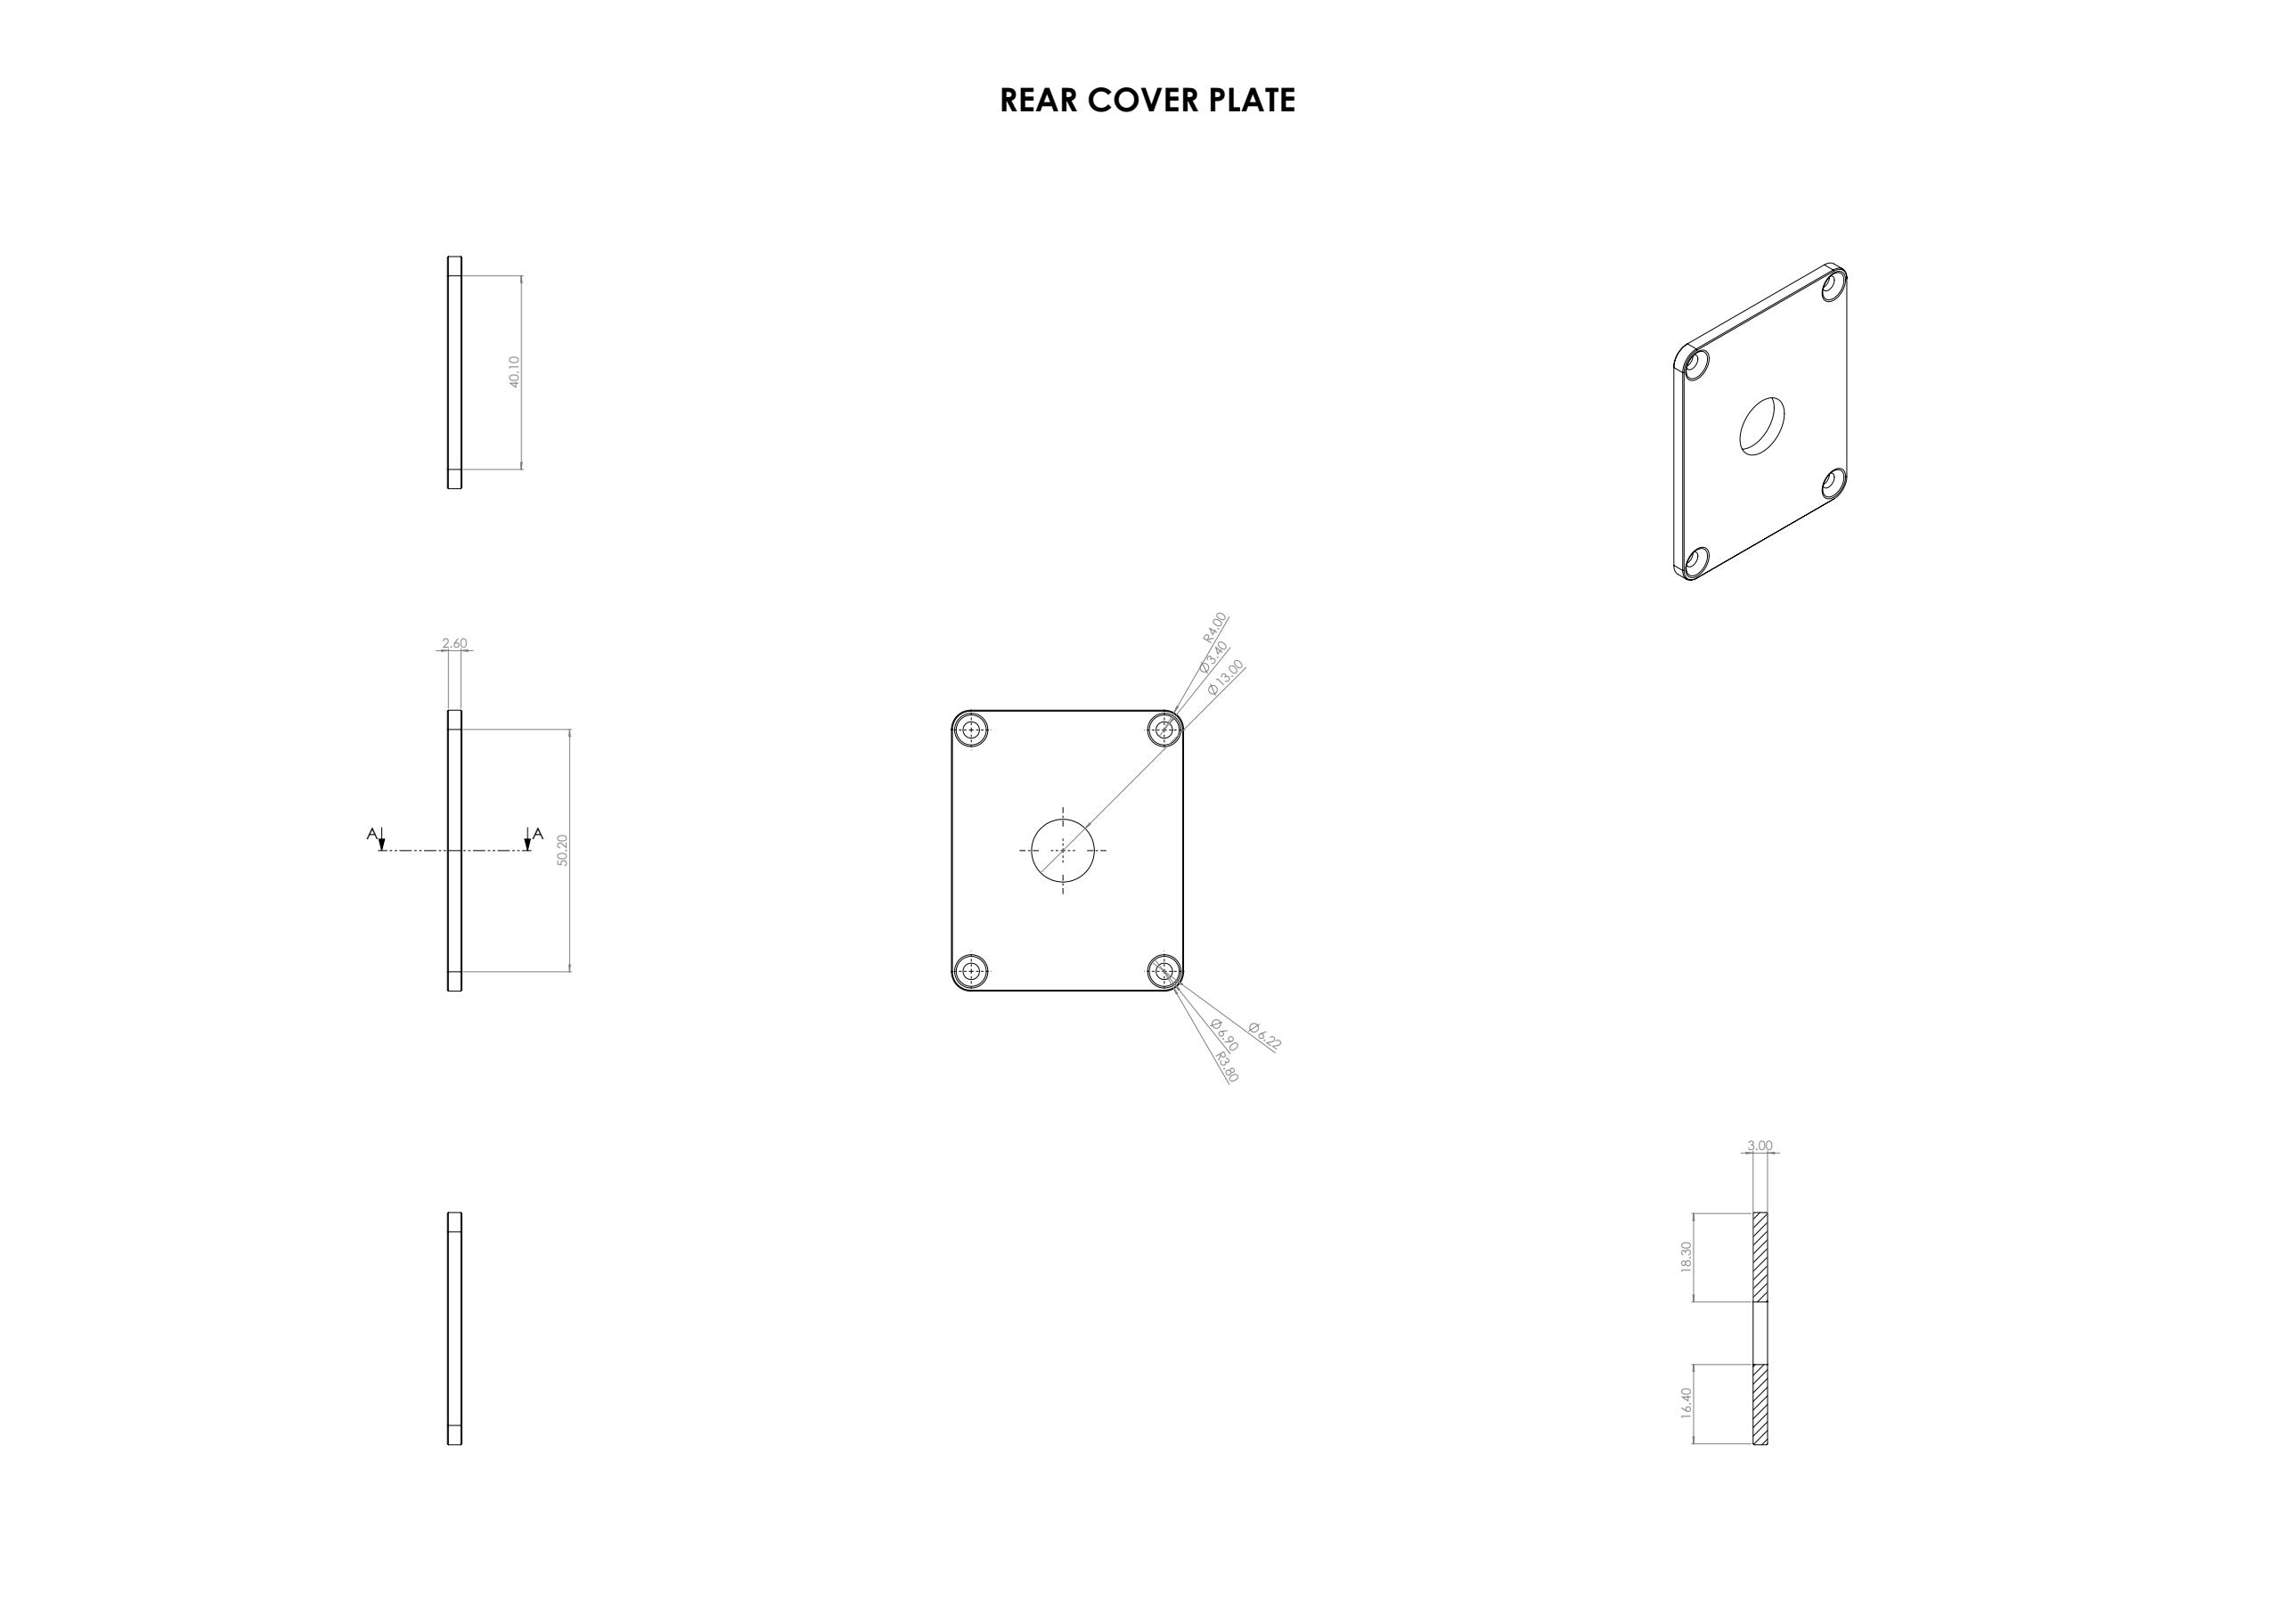
ISO-10303-21;
HEADER;
/* Generated by software containing ST-Developer
 * from STEP Tools, Inc. (www.steptools.com) 
 */

FILE_DESCRIPTION(
/* description */ (''),
/* implementation_level */ '2;1');

FILE_NAME(
/* name */ '07_Rear_Cover_Plate.step',
/* time_stamp */ '2026-10-21T01:59:45-07:00',
/* author */ (''),
/* organization */ (''),
/* preprocessor_version */ 'ST-DEVELOPER v20.2',
/* originating_system */ 'Autodesk Translation Framework v15.15.0.0',
/* authorisation */ '');

FILE_SCHEMA (('AUTOMOTIVE_DESIGN { 1 0 10303 214 3 1 1 }'));
ENDSEC;

DATA;
#10=MECHANICAL_DESIGN_GEOMETRIC_PRESENTATION_REPRESENTATION('',(#466),#18281);
#392=CONICAL_SURFACE('',#9472,3.9,0.78539816339746);
#393=CONICAL_SURFACE('',#9476,3.9,0.785398163397461);
#394=CONICAL_SURFACE('',#9480,3.9,0.785398163397455);
#395=CONICAL_SURFACE('',#9484,3.9,0.785398163397455);
#396=CONICAL_SURFACE('',#9499,3.27928932188134,1.17809724509612);
#397=CONICAL_SURFACE('',#9511,2.475,0.785398163397451);
#398=CONICAL_SURFACE('',#9514,3.9,0.785398163397461);
#399=CONICAL_SURFACE('',#9517,3.9,0.785398163397455);
#400=CONICAL_SURFACE('',#9519,3.9,0.785398163397455);
#401=CONICAL_SURFACE('',#9521,3.9,0.78539816339746);
#402=CONICAL_SURFACE('',#9526,3.27928932188135,1.17809724509617);
#403=CONICAL_SURFACE('',#9528,2.475,0.78539816339745);
#404=CONICAL_SURFACE('',#9530,3.27928932188135,1.17809724509617);
#405=CONICAL_SURFACE('',#9532,2.475,0.78539816339745);
#406=CONICAL_SURFACE('',#9534,3.27928932188134,1.17809724509612);
#407=CONICAL_SURFACE('',#9536,2.475,0.785398163397451);
#440=SHAPE_REPRESENTATION_RELATIONSHIP('SRR','None',#18342,#453);
#453=ADVANCED_BREP_SHAPE_REPRESENTATION('',(#484),#18271);
#466=STYLED_ITEM('',(#18467),#484);
#484=MANIFOLD_SOLID_BREP('Body1',#9088);
#508=CYLINDRICAL_SURFACE('',#9487,4.);
#509=CYLINDRICAL_SURFACE('',#9490,4.);
#510=CYLINDRICAL_SURFACE('',#9524,4.);
#511=CYLINDRICAL_SURFACE('',#9538,1.7);
#512=CYLINDRICAL_SURFACE('',#9539,1.7);
#513=CYLINDRICAL_SURFACE('',#9540,1.7);
#514=CYLINDRICAL_SURFACE('',#9541,1.7);
#515=CYLINDRICAL_SURFACE('',#9542,6.5);
#516=CYLINDRICAL_SURFACE('',#9543,4.);
#598=FACE_BOUND('',#1602,.T.);
#599=FACE_BOUND('',#1603,.T.);
#600=FACE_BOUND('',#1604,.T.);
#601=FACE_BOUND('',#1605,.T.);
#602=FACE_BOUND('',#1606,.T.);
#603=FACE_BOUND('',#1609,.T.);
#604=FACE_BOUND('',#1610,.T.);
#605=FACE_BOUND('',#1611,.T.);
#606=FACE_BOUND('',#1612,.T.);
#607=FACE_BOUND('',#1613,.T.);
#679=CIRCLE('',#9473,4.);
#680=CIRCLE('',#9474,3.8);
#681=CIRCLE('',#9477,4.);
#682=CIRCLE('',#9478,3.8);
#683=CIRCLE('',#9481,4.);
#684=CIRCLE('',#9482,3.8);
#685=CIRCLE('',#9485,4.);
#686=CIRCLE('',#9486,3.8);
#687=CIRCLE('',#9488,4.);
#688=CIRCLE('',#9491,4.);
#689=CIRCLE('',#9494,1.7);
#690=CIRCLE('',#9495,1.7);
#691=CIRCLE('',#9496,1.7);
#692=CIRCLE('',#9497,1.7);
#693=CIRCLE('',#9498,6.5);
#694=CIRCLE('',#9500,3.1085786437627);
#695=CIRCLE('',#9501,3.44999999999999);
#696=CIRCLE('',#9503,3.8);
#697=CIRCLE('',#9504,3.8);
#698=CIRCLE('',#9505,3.8);
#699=CIRCLE('',#9506,3.8);
#700=CIRCLE('',#9507,3.45);
#701=CIRCLE('',#9508,6.5);
#702=CIRCLE('',#9509,3.44999999999999);
#703=CIRCLE('',#9510,3.45);
#704=CIRCLE('',#9512,1.7);
#705=CIRCLE('',#9515,4.);
#706=CIRCLE('',#9522,4.);
#707=CIRCLE('',#9527,3.1085786437627);
#708=CIRCLE('',#9529,1.7);
#709=CIRCLE('',#9531,3.1085786437627);
#710=CIRCLE('',#9533,1.7);
#711=CIRCLE('',#9535,3.1085786437627);
#712=CIRCLE('',#9537,1.7);
#1048=FACE_OUTER_BOUND('',#1589,.T.);
#1049=FACE_OUTER_BOUND('',#1590,.T.);
#1050=FACE_OUTER_BOUND('',#1591,.T.);
#1051=FACE_OUTER_BOUND('',#1592,.T.);
#1052=FACE_OUTER_BOUND('',#1593,.T.);
#1053=FACE_OUTER_BOUND('',#1594,.T.);
#1054=FACE_OUTER_BOUND('',#1595,.T.);
#1055=FACE_OUTER_BOUND('',#1596,.T.);
#1056=FACE_OUTER_BOUND('',#1597,.T.);
#1057=FACE_OUTER_BOUND('',#1598,.T.);
#1058=FACE_OUTER_BOUND('',#1599,.T.);
#1059=FACE_OUTER_BOUND('',#1600,.T.);
#1060=FACE_OUTER_BOUND('',#1601,.T.);
#1061=FACE_OUTER_BOUND('',#1607,.T.);
#1062=FACE_OUTER_BOUND('',#1608,.T.);
#1063=FACE_OUTER_BOUND('',#1614,.T.);
#1064=FACE_OUTER_BOUND('',#1615,.T.);
#1065=FACE_OUTER_BOUND('',#1616,.T.);
#1066=FACE_OUTER_BOUND('',#1617,.T.);
#1067=FACE_OUTER_BOUND('',#1618,.T.);
#1068=FACE_OUTER_BOUND('',#1619,.T.);
#1069=FACE_OUTER_BOUND('',#1620,.T.);
#1070=FACE_OUTER_BOUND('',#1621,.T.);
#1071=FACE_OUTER_BOUND('',#1622,.T.);
#1072=FACE_OUTER_BOUND('',#1623,.T.);
#1073=FACE_OUTER_BOUND('',#1624,.T.);
#1074=FACE_OUTER_BOUND('',#1625,.T.);
#1075=FACE_OUTER_BOUND('',#1626,.T.);
#1076=FACE_OUTER_BOUND('',#1627,.T.);
#1077=FACE_OUTER_BOUND('',#1628,.T.);
#1078=FACE_OUTER_BOUND('',#1629,.T.);
#1079=FACE_OUTER_BOUND('',#1630,.T.);
#1080=FACE_OUTER_BOUND('',#1631,.T.);
#1081=FACE_OUTER_BOUND('',#1632,.T.);
#1082=FACE_OUTER_BOUND('',#1633,.T.);
#1083=FACE_OUTER_BOUND('',#1634,.T.);
#1084=FACE_OUTER_BOUND('',#1635,.T.);
#1085=FACE_OUTER_BOUND('',#1636,.T.);
#1086=FACE_OUTER_BOUND('',#1637,.T.);
#1589=EDGE_LOOP('',(#6750,#6751,#6752,#6753));
#1590=EDGE_LOOP('',(#6754,#6755,#6756,#6757));
#1591=EDGE_LOOP('',(#6758,#6759,#6760,#6761));
#1592=EDGE_LOOP('',(#6762,#6763,#6764,#6765));
#1593=EDGE_LOOP('',(#6766,#6767,#6768,#6769));
#1594=EDGE_LOOP('',(#6770,#6771,#6772,#6773));
#1595=EDGE_LOOP('',(#6774,#6775,#6776,#6777));
#1596=EDGE_LOOP('',(#6778,#6779,#6780,#6781));
#1597=EDGE_LOOP('',(#6782,#6783,#6784,#6785));
#1598=EDGE_LOOP('',(#6786,#6787,#6788,#6789));
#1599=EDGE_LOOP('',(#6790,#6791,#6792,#6793));
#1600=EDGE_LOOP('',(#6794,#6795,#6796,#6797));
#1601=EDGE_LOOP('',(#6798,#6799,#6800,#6801,#6802,#6803,#6804,#6805));
#1602=EDGE_LOOP('',(#6806));
#1603=EDGE_LOOP('',(#6807));
#1604=EDGE_LOOP('',(#6808));
#1605=EDGE_LOOP('',(#6809));
#1606=EDGE_LOOP('',(#6810));
#1607=EDGE_LOOP('',(#6811,#6812,#6813,#6814));
#1608=EDGE_LOOP('',(#6815,#6816,#6817,#6818,#6819,#6820,#6821,#6822));
#1609=EDGE_LOOP('',(#6823));
#1610=EDGE_LOOP('',(#6824));
#1611=EDGE_LOOP('',(#6825));
#1612=EDGE_LOOP('',(#6826));
#1613=EDGE_LOOP('',(#6827));
#1614=EDGE_LOOP('',(#6828,#6829,#6830,#6831));
#1615=EDGE_LOOP('',(#6832,#6833,#6834,#6835));
#1616=EDGE_LOOP('',(#6836,#6837,#6838,#6839));
#1617=EDGE_LOOP('',(#6840,#6841,#6842,#6843));
#1618=EDGE_LOOP('',(#6844,#6845,#6846,#6847));
#1619=EDGE_LOOP('',(#6848,#6849,#6850,#6851));
#1620=EDGE_LOOP('',(#6852,#6853,#6854,#6855));
#1621=EDGE_LOOP('',(#6856,#6857,#6858,#6859));
#1622=EDGE_LOOP('',(#6860,#6861,#6862,#6863));
#1623=EDGE_LOOP('',(#6864,#6865,#6866,#6867));
#1624=EDGE_LOOP('',(#6868,#6869,#6870,#6871));
#1625=EDGE_LOOP('',(#6872,#6873,#6874,#6875));
#1626=EDGE_LOOP('',(#6876,#6877,#6878,#6879));
#1627=EDGE_LOOP('',(#6880,#6881,#6882,#6883));
#1628=EDGE_LOOP('',(#6884,#6885,#6886,#6887));
#1629=EDGE_LOOP('',(#6888,#6889,#6890,#6891));
#1630=EDGE_LOOP('',(#6892,#6893,#6894,#6895));
#1631=EDGE_LOOP('',(#6896,#6897,#6898,#6899));
#1632=EDGE_LOOP('',(#6900,#6901,#6902,#6903));
#1633=EDGE_LOOP('',(#6904,#6905,#6906,#6907));
#1634=EDGE_LOOP('',(#6908,#6909,#6910,#6911));
#1635=EDGE_LOOP('',(#6912,#6913,#6914,#6915));
#1636=EDGE_LOOP('',(#6916,#6917,#6918,#6919));
#1637=EDGE_LOOP('',(#6920,#6921,#6922,#6923));
#2304=LINE('',#13823,#3149);
#2305=LINE('',#13825,#3150);
#2306=LINE('',#13827,#3151);
#2307=LINE('',#13828,#3152);
#2308=LINE('',#13832,#3153);
#2309=LINE('',#13838,#3154);
#2310=LINE('',#13839,#3155);
#2311=LINE('',#13840,#3156);
#2312=LINE('',#13844,#3157);
#2313=LINE('',#13850,#3158);
#2314=LINE('',#13851,#3159);
#2315=LINE('',#13852,#3160);
#2316=LINE('',#13856,#3161);
#2317=LINE('',#13862,#3162);
#2318=LINE('',#13863,#3163);
#2319=LINE('',#13864,#3164);
#2320=LINE('',#13870,#3165);
#2321=LINE('',#13873,#3166);
#2322=LINE('',#13876,#3167);
#2323=LINE('',#13877,#3168);
#2324=LINE('',#13880,#3169);
#2325=LINE('',#13884,#3170);
#2326=LINE('',#13885,#3171);
#2327=LINE('',#13901,#3172);
#2328=LINE('',#13906,#3173);
#2329=LINE('',#13910,#3174);
#2330=LINE('',#13914,#3175);
#2331=LINE('',#13918,#3176);
#2332=LINE('',#13930,#3177);
#2333=LINE('',#13934,#3178);
#2334=LINE('',#13936,#3179);
#2335=LINE('',#13937,#3180);
#2336=LINE('',#13941,#3181);
#2337=LINE('',#13943,#3182);
#2338=LINE('',#13944,#3183);
#2339=LINE('',#13946,#3184);
#2340=LINE('',#13948,#3185);
#2341=LINE('',#13950,#3186);
#2342=LINE('',#13952,#3187);
#2343=LINE('',#13956,#3188);
#2344=LINE('',#13958,#3189);
#2345=LINE('',#13960,#3190);
#2346=LINE('',#13964,#3191);
#2347=LINE('',#13967,#3192);
#2348=LINE('',#13972,#3193);
#2349=LINE('',#13975,#3194);
#2350=LINE('',#13980,#3195);
#2351=LINE('',#13983,#3196);
#2352=LINE('',#13986,#3197);
#2353=LINE('',#13988,#3198);
#2354=LINE('',#13990,#3199);
#2355=LINE('',#13992,#3200);
#2356=LINE('',#13994,#3201);
#3149=VECTOR('',#10798,10.);
#3150=VECTOR('',#10799,10.);
#3151=VECTOR('',#10800,10.);
#3152=VECTOR('',#10801,10.);
#3153=VECTOR('',#10804,10.);
#3154=VECTOR('',#10811,10.);
#3155=VECTOR('',#10812,10.);
#3156=VECTOR('',#10813,10.);
#3157=VECTOR('',#10816,10.);
#3158=VECTOR('',#10823,10.);
#3159=VECTOR('',#10824,10.);
#3160=VECTOR('',#10825,10.);
#3161=VECTOR('',#10828,10.);
#3162=VECTOR('',#10835,10.);
#3163=VECTOR('',#10836,10.);
#3164=VECTOR('',#10837,10.);
#3165=VECTOR('',#10846,10.);
#3166=VECTOR('',#10849,10.);
#3167=VECTOR('',#10852,10.);
#3168=VECTOR('',#10853,10.);
#3169=VECTOR('',#10856,10.);
#3170=VECTOR('',#10861,10.);
#3171=VECTOR('',#10862,10.);
#3172=VECTOR('',#10879,3.27928932188134);
#3173=VECTOR('',#10884,10.);
#3174=VECTOR('',#10887,10.);
#3175=VECTOR('',#10890,10.);
#3176=VECTOR('',#10893,10.);
#3177=VECTOR('',#10906,2.475);
#3178=VECTOR('',#10911,10.);
#3179=VECTOR('',#10912,10.);
#3180=VECTOR('',#10913,10.);
#3181=VECTOR('',#10918,10.);
#3182=VECTOR('',#10921,10.);
#3183=VECTOR('',#10922,10.);
#3184=VECTOR('',#10925,10.);
#3185=VECTOR('',#10928,10.);
#3186=VECTOR('',#10931,10.);
#3187=VECTOR('',#10934,10.);
#3188=VECTOR('',#10941,10.);
#3189=VECTOR('',#10944,10.);
#3190=VECTOR('',#10947,10.);
#3191=VECTOR('',#10952,3.27928932188135);
#3192=VECTOR('',#10955,2.475);
#3193=VECTOR('',#10962,3.27928932188135);
#3194=VECTOR('',#10965,2.475);
#3195=VECTOR('',#10972,3.27928932188134);
#3196=VECTOR('',#10975,2.475);
#3197=VECTOR('',#10980,1.7);
#3198=VECTOR('',#10983,1.7);
#3199=VECTOR('',#10986,1.7);
#3200=VECTOR('',#10989,1.7);
#3201=VECTOR('',#10992,6.5);
#3958=VERTEX_POINT('',#13821);
#3959=VERTEX_POINT('',#13822);
#3960=VERTEX_POINT('',#13824);
#3961=VERTEX_POINT('',#13826);
#3962=VERTEX_POINT('',#13830);
#3963=VERTEX_POINT('',#13831);
#3964=VERTEX_POINT('',#13836);
#3965=VERTEX_POINT('',#13837);
#3966=VERTEX_POINT('',#13842);
#3967=VERTEX_POINT('',#13843);
#3968=VERTEX_POINT('',#13848);
#3969=VERTEX_POINT('',#13849);
#3970=VERTEX_POINT('',#13854);
#3971=VERTEX_POINT('',#13855);
#3972=VERTEX_POINT('',#13860);
#3973=VERTEX_POINT('',#13861);
#3974=VERTEX_POINT('',#13869);
#3975=VERTEX_POINT('',#13871);
#3976=VERTEX_POINT('',#13875);
#3977=VERTEX_POINT('',#13879);
#3978=VERTEX_POINT('',#13883);
#3979=VERTEX_POINT('',#13887);
#3980=VERTEX_POINT('',#13889);
#3981=VERTEX_POINT('',#13891);
#3982=VERTEX_POINT('',#13893);
#3983=VERTEX_POINT('',#13895);
#3984=VERTEX_POINT('',#13898);
#3985=VERTEX_POINT('',#13900);
#3986=VERTEX_POINT('',#13904);
#3987=VERTEX_POINT('',#13905);
#3988=VERTEX_POINT('',#13907);
#3989=VERTEX_POINT('',#13909);
#3990=VERTEX_POINT('',#13911);
#3991=VERTEX_POINT('',#13913);
#3992=VERTEX_POINT('',#13915);
#3993=VERTEX_POINT('',#13917);
#3994=VERTEX_POINT('',#13920);
#3995=VERTEX_POINT('',#13922);
#3996=VERTEX_POINT('',#13924);
#3997=VERTEX_POINT('',#13926);
#3998=VERTEX_POINT('',#13929);
#3999=VERTEX_POINT('',#13933);
#4000=VERTEX_POINT('',#13935);
#4001=VERTEX_POINT('',#13939);
#4002=VERTEX_POINT('',#13962);
#4003=VERTEX_POINT('',#13966);
#4004=VERTEX_POINT('',#13970);
#4005=VERTEX_POINT('',#13974);
#4006=VERTEX_POINT('',#13978);
#4007=VERTEX_POINT('',#13982);
#4947=EDGE_CURVE('',#3958,#3959,#2304,.T.);
#4948=EDGE_CURVE('',#3959,#3960,#2305,.T.);
#4949=EDGE_CURVE('',#3960,#3961,#2306,.T.);
#4950=EDGE_CURVE('',#3961,#3958,#2307,.T.);
#4951=EDGE_CURVE('',#3962,#3963,#2308,.T.);
#4952=EDGE_CURVE('',#3963,#3959,#679,.T.);
#4953=EDGE_CURVE('',#3958,#3962,#680,.T.);
#4954=EDGE_CURVE('',#3964,#3965,#2309,.T.);
#4955=EDGE_CURVE('',#3965,#3963,#2310,.T.);
#4956=EDGE_CURVE('',#3962,#3964,#2311,.T.);
#4957=EDGE_CURVE('',#3966,#3967,#2312,.T.);
#4958=EDGE_CURVE('',#3967,#3965,#681,.T.);
#4959=EDGE_CURVE('',#3964,#3966,#682,.T.);
#4960=EDGE_CURVE('',#3968,#3969,#2313,.T.);
#4961=EDGE_CURVE('',#3969,#3967,#2314,.T.);
#4962=EDGE_CURVE('',#3966,#3968,#2315,.T.);
#4963=EDGE_CURVE('',#3970,#3971,#2316,.T.);
#4964=EDGE_CURVE('',#3971,#3969,#683,.T.);
#4965=EDGE_CURVE('',#3968,#3970,#684,.T.);
#4966=EDGE_CURVE('',#3972,#3973,#2317,.T.);
#4967=EDGE_CURVE('',#3973,#3971,#2318,.T.);
#4968=EDGE_CURVE('',#3970,#3972,#2319,.T.);
#4969=EDGE_CURVE('',#3960,#3973,#685,.T.);
#4970=EDGE_CURVE('',#3972,#3961,#686,.T.);
#4971=EDGE_CURVE('',#3971,#3974,#2320,.T.);
#4972=EDGE_CURVE('',#3975,#3974,#687,.T.);
#4973=EDGE_CURVE('',#3975,#3969,#2321,.T.);
#4974=EDGE_CURVE('',#3976,#3973,#2322,.T.);
#4975=EDGE_CURVE('',#3974,#3976,#2323,.T.);
#4976=EDGE_CURVE('',#3960,#3977,#2324,.T.);
#4977=EDGE_CURVE('',#3976,#3977,#688,.T.);
#4978=EDGE_CURVE('',#3978,#3959,#2325,.T.);
#4979=EDGE_CURVE('',#3977,#3978,#2326,.T.);
#4980=EDGE_CURVE('',#3979,#3979,#689,.T.);
#4981=EDGE_CURVE('',#3980,#3980,#690,.T.);
#4982=EDGE_CURVE('',#3981,#3981,#691,.T.);
#4983=EDGE_CURVE('',#3982,#3982,#692,.T.);
#4984=EDGE_CURVE('',#3983,#3983,#693,.T.);
#4985=EDGE_CURVE('',#3984,#3984,#694,.T.);
#4986=EDGE_CURVE('',#3984,#3985,#2327,.T.);
#4987=EDGE_CURVE('',#3985,#3985,#695,.T.);
#4988=EDGE_CURVE('',#3986,#3987,#2328,.T.);
#4989=EDGE_CURVE('',#3988,#3986,#696,.T.);
#4990=EDGE_CURVE('',#3989,#3988,#2329,.T.);
#4991=EDGE_CURVE('',#3990,#3989,#697,.T.);
#4992=EDGE_CURVE('',#3991,#3990,#2330,.T.);
#4993=EDGE_CURVE('',#3992,#3991,#698,.T.);
#4994=EDGE_CURVE('',#3993,#3992,#2331,.T.);
#4995=EDGE_CURVE('',#3987,#3993,#699,.T.);
#4996=EDGE_CURVE('',#3994,#3994,#700,.T.);
#4997=EDGE_CURVE('',#3995,#3995,#701,.T.);
#4998=EDGE_CURVE('',#3996,#3996,#702,.T.);
#4999=EDGE_CURVE('',#3997,#3997,#703,.T.);
#5000=EDGE_CURVE('',#3984,#3998,#2332,.T.);
#5001=EDGE_CURVE('',#3998,#3998,#704,.T.);
#5002=EDGE_CURVE('',#3999,#3986,#2333,.T.);
#5003=EDGE_CURVE('',#3987,#4000,#2334,.T.);
#5004=EDGE_CURVE('',#4000,#3999,#2335,.T.);
#5005=EDGE_CURVE('',#3999,#4001,#705,.T.);
#5006=EDGE_CURVE('',#4001,#3988,#2336,.T.);
#5007=EDGE_CURVE('',#3975,#3989,#2337,.T.);
#5008=EDGE_CURVE('',#4001,#3975,#2338,.T.);
#5009=EDGE_CURVE('',#3974,#3990,#2339,.T.);
#5010=EDGE_CURVE('',#3976,#3991,#2340,.T.);
#5011=EDGE_CURVE('',#3977,#3992,#2341,.T.);
#5012=EDGE_CURVE('',#3978,#3993,#2342,.T.);
#5013=EDGE_CURVE('',#3978,#4000,#706,.T.);
#5014=EDGE_CURVE('',#3967,#4001,#2343,.T.);
#5015=EDGE_CURVE('',#3999,#3965,#2344,.T.);
#5016=EDGE_CURVE('',#3963,#4000,#2345,.T.);
#5017=EDGE_CURVE('',#4002,#4002,#707,.T.);
#5018=EDGE_CURVE('',#4002,#3997,#2346,.T.);
#5019=EDGE_CURVE('',#4002,#4003,#2347,.T.);
#5020=EDGE_CURVE('',#4003,#4003,#708,.T.);
#5021=EDGE_CURVE('',#4004,#4004,#709,.T.);
#5022=EDGE_CURVE('',#4004,#3994,#2348,.T.);
#5023=EDGE_CURVE('',#4004,#4005,#2349,.T.);
#5024=EDGE_CURVE('',#4005,#4005,#710,.T.);
#5025=EDGE_CURVE('',#4006,#4006,#711,.T.);
#5026=EDGE_CURVE('',#4006,#3996,#2350,.T.);
#5027=EDGE_CURVE('',#4006,#4007,#2351,.T.);
#5028=EDGE_CURVE('',#4007,#4007,#712,.T.);
#5029=EDGE_CURVE('',#4007,#3982,#2352,.T.);
#5030=EDGE_CURVE('',#4005,#3981,#2353,.T.);
#5031=EDGE_CURVE('',#3998,#3980,#2354,.T.);
#5032=EDGE_CURVE('',#4003,#3979,#2355,.T.);
#5033=EDGE_CURVE('',#3995,#3983,#2356,.T.);
#6750=ORIENTED_EDGE('',*,*,#4947,.T.);
#6751=ORIENTED_EDGE('',*,*,#4948,.T.);
#6752=ORIENTED_EDGE('',*,*,#4949,.T.);
#6753=ORIENTED_EDGE('',*,*,#4950,.T.);
#6754=ORIENTED_EDGE('',*,*,#4951,.T.);
#6755=ORIENTED_EDGE('',*,*,#4952,.T.);
#6756=ORIENTED_EDGE('',*,*,#4947,.F.);
#6757=ORIENTED_EDGE('',*,*,#4953,.T.);
#6758=ORIENTED_EDGE('',*,*,#4954,.T.);
#6759=ORIENTED_EDGE('',*,*,#4955,.T.);
#6760=ORIENTED_EDGE('',*,*,#4951,.F.);
#6761=ORIENTED_EDGE('',*,*,#4956,.T.);
#6762=ORIENTED_EDGE('',*,*,#4957,.T.);
#6763=ORIENTED_EDGE('',*,*,#4958,.T.);
#6764=ORIENTED_EDGE('',*,*,#4954,.F.);
#6765=ORIENTED_EDGE('',*,*,#4959,.T.);
#6766=ORIENTED_EDGE('',*,*,#4960,.T.);
#6767=ORIENTED_EDGE('',*,*,#4961,.T.);
#6768=ORIENTED_EDGE('',*,*,#4957,.F.);
#6769=ORIENTED_EDGE('',*,*,#4962,.T.);
#6770=ORIENTED_EDGE('',*,*,#4963,.T.);
#6771=ORIENTED_EDGE('',*,*,#4964,.T.);
#6772=ORIENTED_EDGE('',*,*,#4960,.F.);
#6773=ORIENTED_EDGE('',*,*,#4965,.T.);
#6774=ORIENTED_EDGE('',*,*,#4966,.T.);
#6775=ORIENTED_EDGE('',*,*,#4967,.T.);
#6776=ORIENTED_EDGE('',*,*,#4963,.F.);
#6777=ORIENTED_EDGE('',*,*,#4968,.T.);
#6778=ORIENTED_EDGE('',*,*,#4949,.F.);
#6779=ORIENTED_EDGE('',*,*,#4969,.T.);
#6780=ORIENTED_EDGE('',*,*,#4966,.F.);
#6781=ORIENTED_EDGE('',*,*,#4970,.T.);
#6782=ORIENTED_EDGE('',*,*,#4964,.F.);
#6783=ORIENTED_EDGE('',*,*,#4971,.T.);
#6784=ORIENTED_EDGE('',*,*,#4972,.F.);
#6785=ORIENTED_EDGE('',*,*,#4973,.T.);
#6786=ORIENTED_EDGE('',*,*,#4967,.F.);
#6787=ORIENTED_EDGE('',*,*,#4974,.F.);
#6788=ORIENTED_EDGE('',*,*,#4975,.F.);
#6789=ORIENTED_EDGE('',*,*,#4971,.F.);
#6790=ORIENTED_EDGE('',*,*,#4969,.F.);
#6791=ORIENTED_EDGE('',*,*,#4976,.T.);
#6792=ORIENTED_EDGE('',*,*,#4977,.F.);
#6793=ORIENTED_EDGE('',*,*,#4974,.T.);
#6794=ORIENTED_EDGE('',*,*,#4948,.F.);
#6795=ORIENTED_EDGE('',*,*,#4978,.F.);
#6796=ORIENTED_EDGE('',*,*,#4979,.F.);
#6797=ORIENTED_EDGE('',*,*,#4976,.F.);
#6798=ORIENTED_EDGE('',*,*,#4950,.F.);
#6799=ORIENTED_EDGE('',*,*,#4970,.F.);
#6800=ORIENTED_EDGE('',*,*,#4968,.F.);
#6801=ORIENTED_EDGE('',*,*,#4965,.F.);
#6802=ORIENTED_EDGE('',*,*,#4962,.F.);
#6803=ORIENTED_EDGE('',*,*,#4959,.F.);
#6804=ORIENTED_EDGE('',*,*,#4956,.F.);
#6805=ORIENTED_EDGE('',*,*,#4953,.F.);
#6806=ORIENTED_EDGE('',*,*,#4980,.T.);
#6807=ORIENTED_EDGE('',*,*,#4981,.T.);
#6808=ORIENTED_EDGE('',*,*,#4982,.T.);
#6809=ORIENTED_EDGE('',*,*,#4983,.T.);
#6810=ORIENTED_EDGE('',*,*,#4984,.T.);
#6811=ORIENTED_EDGE('',*,*,#4985,.T.);
#6812=ORIENTED_EDGE('',*,*,#4986,.T.);
#6813=ORIENTED_EDGE('',*,*,#4987,.T.);
#6814=ORIENTED_EDGE('',*,*,#4986,.F.);
#6815=ORIENTED_EDGE('',*,*,#4988,.F.);
#6816=ORIENTED_EDGE('',*,*,#4989,.F.);
#6817=ORIENTED_EDGE('',*,*,#4990,.F.);
#6818=ORIENTED_EDGE('',*,*,#4991,.F.);
#6819=ORIENTED_EDGE('',*,*,#4992,.F.);
#6820=ORIENTED_EDGE('',*,*,#4993,.F.);
#6821=ORIENTED_EDGE('',*,*,#4994,.F.);
#6822=ORIENTED_EDGE('',*,*,#4995,.F.);
#6823=ORIENTED_EDGE('',*,*,#4996,.F.);
#6824=ORIENTED_EDGE('',*,*,#4997,.T.);
#6825=ORIENTED_EDGE('',*,*,#4998,.F.);
#6826=ORIENTED_EDGE('',*,*,#4999,.F.);
#6827=ORIENTED_EDGE('',*,*,#4987,.F.);
#6828=ORIENTED_EDGE('',*,*,#4985,.F.);
#6829=ORIENTED_EDGE('',*,*,#5000,.T.);
#6830=ORIENTED_EDGE('',*,*,#5001,.T.);
#6831=ORIENTED_EDGE('',*,*,#5000,.F.);
#6832=ORIENTED_EDGE('',*,*,#5002,.T.);
#6833=ORIENTED_EDGE('',*,*,#4988,.T.);
#6834=ORIENTED_EDGE('',*,*,#5003,.T.);
#6835=ORIENTED_EDGE('',*,*,#5004,.T.);
#6836=ORIENTED_EDGE('',*,*,#5002,.F.);
#6837=ORIENTED_EDGE('',*,*,#5005,.T.);
#6838=ORIENTED_EDGE('',*,*,#5006,.T.);
#6839=ORIENTED_EDGE('',*,*,#4989,.T.);
#6840=ORIENTED_EDGE('',*,*,#5007,.T.);
#6841=ORIENTED_EDGE('',*,*,#4990,.T.);
#6842=ORIENTED_EDGE('',*,*,#5006,.F.);
#6843=ORIENTED_EDGE('',*,*,#5008,.T.);
#6844=ORIENTED_EDGE('',*,*,#5007,.F.);
#6845=ORIENTED_EDGE('',*,*,#4972,.T.);
#6846=ORIENTED_EDGE('',*,*,#5009,.T.);
#6847=ORIENTED_EDGE('',*,*,#4991,.T.);
#6848=ORIENTED_EDGE('',*,*,#5010,.T.);
#6849=ORIENTED_EDGE('',*,*,#4992,.T.);
#6850=ORIENTED_EDGE('',*,*,#5009,.F.);
#6851=ORIENTED_EDGE('',*,*,#4975,.T.);
#6852=ORIENTED_EDGE('',*,*,#5010,.F.);
#6853=ORIENTED_EDGE('',*,*,#4977,.T.);
#6854=ORIENTED_EDGE('',*,*,#5011,.T.);
#6855=ORIENTED_EDGE('',*,*,#4993,.T.);
#6856=ORIENTED_EDGE('',*,*,#5012,.T.);
#6857=ORIENTED_EDGE('',*,*,#4994,.T.);
#6858=ORIENTED_EDGE('',*,*,#5011,.F.);
#6859=ORIENTED_EDGE('',*,*,#4979,.T.);
#6860=ORIENTED_EDGE('',*,*,#5012,.F.);
#6861=ORIENTED_EDGE('',*,*,#5013,.T.);
#6862=ORIENTED_EDGE('',*,*,#5003,.F.);
#6863=ORIENTED_EDGE('',*,*,#4995,.T.);
#6864=ORIENTED_EDGE('',*,*,#4961,.F.);
#6865=ORIENTED_EDGE('',*,*,#4973,.F.);
#6866=ORIENTED_EDGE('',*,*,#5008,.F.);
#6867=ORIENTED_EDGE('',*,*,#5014,.F.);
#6868=ORIENTED_EDGE('',*,*,#4958,.F.);
#6869=ORIENTED_EDGE('',*,*,#5014,.T.);
#6870=ORIENTED_EDGE('',*,*,#5005,.F.);
#6871=ORIENTED_EDGE('',*,*,#5015,.T.);
#6872=ORIENTED_EDGE('',*,*,#4955,.F.);
#6873=ORIENTED_EDGE('',*,*,#5015,.F.);
#6874=ORIENTED_EDGE('',*,*,#5004,.F.);
#6875=ORIENTED_EDGE('',*,*,#5016,.F.);
#6876=ORIENTED_EDGE('',*,*,#5017,.T.);
#6877=ORIENTED_EDGE('',*,*,#5018,.T.);
#6878=ORIENTED_EDGE('',*,*,#4999,.T.);
#6879=ORIENTED_EDGE('',*,*,#5018,.F.);
#6880=ORIENTED_EDGE('',*,*,#5017,.F.);
#6881=ORIENTED_EDGE('',*,*,#5019,.T.);
#6882=ORIENTED_EDGE('',*,*,#5020,.T.);
#6883=ORIENTED_EDGE('',*,*,#5019,.F.);
#6884=ORIENTED_EDGE('',*,*,#5021,.T.);
#6885=ORIENTED_EDGE('',*,*,#5022,.T.);
#6886=ORIENTED_EDGE('',*,*,#4996,.T.);
#6887=ORIENTED_EDGE('',*,*,#5022,.F.);
#6888=ORIENTED_EDGE('',*,*,#5021,.F.);
#6889=ORIENTED_EDGE('',*,*,#5023,.T.);
#6890=ORIENTED_EDGE('',*,*,#5024,.T.);
#6891=ORIENTED_EDGE('',*,*,#5023,.F.);
#6892=ORIENTED_EDGE('',*,*,#5025,.T.);
#6893=ORIENTED_EDGE('',*,*,#5026,.T.);
#6894=ORIENTED_EDGE('',*,*,#4998,.T.);
#6895=ORIENTED_EDGE('',*,*,#5026,.F.);
#6896=ORIENTED_EDGE('',*,*,#5025,.F.);
#6897=ORIENTED_EDGE('',*,*,#5027,.T.);
#6898=ORIENTED_EDGE('',*,*,#5028,.T.);
#6899=ORIENTED_EDGE('',*,*,#5027,.F.);
#6900=ORIENTED_EDGE('',*,*,#5028,.F.);
#6901=ORIENTED_EDGE('',*,*,#5029,.T.);
#6902=ORIENTED_EDGE('',*,*,#4983,.F.);
#6903=ORIENTED_EDGE('',*,*,#5029,.F.);
#6904=ORIENTED_EDGE('',*,*,#5024,.F.);
#6905=ORIENTED_EDGE('',*,*,#5030,.T.);
#6906=ORIENTED_EDGE('',*,*,#4982,.F.);
#6907=ORIENTED_EDGE('',*,*,#5030,.F.);
#6908=ORIENTED_EDGE('',*,*,#5001,.F.);
#6909=ORIENTED_EDGE('',*,*,#5031,.T.);
#6910=ORIENTED_EDGE('',*,*,#4981,.F.);
#6911=ORIENTED_EDGE('',*,*,#5031,.F.);
#6912=ORIENTED_EDGE('',*,*,#5020,.F.);
#6913=ORIENTED_EDGE('',*,*,#5032,.T.);
#6914=ORIENTED_EDGE('',*,*,#4980,.F.);
#6915=ORIENTED_EDGE('',*,*,#5032,.F.);
#6916=ORIENTED_EDGE('',*,*,#4997,.F.);
#6917=ORIENTED_EDGE('',*,*,#5033,.T.);
#6918=ORIENTED_EDGE('',*,*,#4984,.F.);
#6919=ORIENTED_EDGE('',*,*,#5033,.F.);
#6920=ORIENTED_EDGE('',*,*,#4952,.F.);
#6921=ORIENTED_EDGE('',*,*,#5016,.T.);
#6922=ORIENTED_EDGE('',*,*,#5013,.F.);
#6923=ORIENTED_EDGE('',*,*,#4978,.T.);
#8368=PLANE('',#9471);
#8369=PLANE('',#9475);
#8370=PLANE('',#9479);
#8371=PLANE('',#9483);
#8372=PLANE('',#9489);
#8373=PLANE('',#9492);
#8374=PLANE('',#9493);
#8375=PLANE('',#9502);
#8376=PLANE('',#9513);
#8377=PLANE('',#9516);
#8378=PLANE('',#9518);
#8379=PLANE('',#9520);
#8380=PLANE('',#9523);
#8381=PLANE('',#9525);
#8769=ADVANCED_FACE('',(#1048),#8368,.T.);
#8770=ADVANCED_FACE('',(#1049),#392,.T.);
#8771=ADVANCED_FACE('',(#1050),#8369,.T.);
#8772=ADVANCED_FACE('',(#1051),#393,.T.);
#8773=ADVANCED_FACE('',(#1052),#8370,.T.);
#8774=ADVANCED_FACE('',(#1053),#394,.T.);
#8775=ADVANCED_FACE('',(#1054),#8371,.T.);
#8776=ADVANCED_FACE('',(#1055),#395,.T.);
#8777=ADVANCED_FACE('',(#1056),#508,.T.);
#8778=ADVANCED_FACE('',(#1057),#8372,.T.);
#8779=ADVANCED_FACE('',(#1058),#509,.T.);
#8780=ADVANCED_FACE('',(#1059),#8373,.T.);
#8781=ADVANCED_FACE('',(#1060,#598,#599,#600,#601,#602),#8374,.F.);
#8782=ADVANCED_FACE('',(#1061),#396,.F.);
#8783=ADVANCED_FACE('',(#1062,#603,#604,#605,#606,#607),#8375,.T.);
#8784=ADVANCED_FACE('',(#1063),#397,.F.);
#8785=ADVANCED_FACE('',(#1064),#8376,.T.);
#8786=ADVANCED_FACE('',(#1065),#398,.T.);
#8787=ADVANCED_FACE('',(#1066),#8377,.T.);
#8788=ADVANCED_FACE('',(#1067),#399,.T.);
#8789=ADVANCED_FACE('',(#1068),#8378,.T.);
#8790=ADVANCED_FACE('',(#1069),#400,.T.);
#8791=ADVANCED_FACE('',(#1070),#8379,.T.);
#8792=ADVANCED_FACE('',(#1071),#401,.T.);
#8793=ADVANCED_FACE('',(#1072),#8380,.T.);
#8794=ADVANCED_FACE('',(#1073),#510,.T.);
#8795=ADVANCED_FACE('',(#1074),#8381,.T.);
#8796=ADVANCED_FACE('',(#1075),#402,.F.);
#8797=ADVANCED_FACE('',(#1076),#403,.F.);
#8798=ADVANCED_FACE('',(#1077),#404,.F.);
#8799=ADVANCED_FACE('',(#1078),#405,.F.);
#8800=ADVANCED_FACE('',(#1079),#406,.F.);
#8801=ADVANCED_FACE('',(#1080),#407,.F.);
#8802=ADVANCED_FACE('',(#1081),#511,.F.);
#8803=ADVANCED_FACE('',(#1082),#512,.F.);
#8804=ADVANCED_FACE('',(#1083),#513,.F.);
#8805=ADVANCED_FACE('',(#1084),#514,.F.);
#8806=ADVANCED_FACE('',(#1085),#515,.F.);
#8807=ADVANCED_FACE('',(#1086),#516,.T.);
#9088=CLOSED_SHELL('',(#8769,#8770,#8771,#8772,#8773,#8774,#8775,#8776,
#8777,#8778,#8779,#8780,#8781,#8782,#8783,#8784,#8785,#8786,#8787,#8788,
#8789,#8790,#8791,#8792,#8793,#8794,#8795,#8796,#8797,#8798,#8799,#8800,
#8801,#8802,#8803,#8804,#8805,#8806,#8807));
#9470=AXIS2_PLACEMENT_3D('',#13819,#10794,#10795);
#9471=AXIS2_PLACEMENT_3D('',#13820,#10796,#10797);
#9472=AXIS2_PLACEMENT_3D('',#13829,#10802,#10803);
#9473=AXIS2_PLACEMENT_3D('',#13833,#10805,#10806);
#9474=AXIS2_PLACEMENT_3D('',#13834,#10807,#10808);
#9475=AXIS2_PLACEMENT_3D('',#13835,#10809,#10810);
#9476=AXIS2_PLACEMENT_3D('',#13841,#10814,#10815);
#9477=AXIS2_PLACEMENT_3D('',#13845,#10817,#10818);
#9478=AXIS2_PLACEMENT_3D('',#13846,#10819,#10820);
#9479=AXIS2_PLACEMENT_3D('',#13847,#10821,#10822);
#9480=AXIS2_PLACEMENT_3D('',#13853,#10826,#10827);
#9481=AXIS2_PLACEMENT_3D('',#13857,#10829,#10830);
#9482=AXIS2_PLACEMENT_3D('',#13858,#10831,#10832);
#9483=AXIS2_PLACEMENT_3D('',#13859,#10833,#10834);
#9484=AXIS2_PLACEMENT_3D('',#13865,#10838,#10839);
#9485=AXIS2_PLACEMENT_3D('',#13866,#10840,#10841);
#9486=AXIS2_PLACEMENT_3D('',#13867,#10842,#10843);
#9487=AXIS2_PLACEMENT_3D('',#13868,#10844,#10845);
#9488=AXIS2_PLACEMENT_3D('',#13872,#10847,#10848);
#9489=AXIS2_PLACEMENT_3D('',#13874,#10850,#10851);
#9490=AXIS2_PLACEMENT_3D('',#13878,#10854,#10855);
#9491=AXIS2_PLACEMENT_3D('',#13881,#10857,#10858);
#9492=AXIS2_PLACEMENT_3D('',#13882,#10859,#10860);
#9493=AXIS2_PLACEMENT_3D('',#13886,#10863,#10864);
#9494=AXIS2_PLACEMENT_3D('',#13888,#10865,#10866);
#9495=AXIS2_PLACEMENT_3D('',#13890,#10867,#10868);
#9496=AXIS2_PLACEMENT_3D('',#13892,#10869,#10870);
#9497=AXIS2_PLACEMENT_3D('',#13894,#10871,#10872);
#9498=AXIS2_PLACEMENT_3D('',#13896,#10873,#10874);
#9499=AXIS2_PLACEMENT_3D('',#13897,#10875,#10876);
#9500=AXIS2_PLACEMENT_3D('',#13899,#10877,#10878);
#9501=AXIS2_PLACEMENT_3D('',#13902,#10880,#10881);
#9502=AXIS2_PLACEMENT_3D('',#13903,#10882,#10883);
#9503=AXIS2_PLACEMENT_3D('',#13908,#10885,#10886);
#9504=AXIS2_PLACEMENT_3D('',#13912,#10888,#10889);
#9505=AXIS2_PLACEMENT_3D('',#13916,#10891,#10892);
#9506=AXIS2_PLACEMENT_3D('',#13919,#10894,#10895);
#9507=AXIS2_PLACEMENT_3D('',#13921,#10896,#10897);
#9508=AXIS2_PLACEMENT_3D('',#13923,#10898,#10899);
#9509=AXIS2_PLACEMENT_3D('',#13925,#10900,#10901);
#9510=AXIS2_PLACEMENT_3D('',#13927,#10902,#10903);
#9511=AXIS2_PLACEMENT_3D('',#13928,#10904,#10905);
#9512=AXIS2_PLACEMENT_3D('',#13931,#10907,#10908);
#9513=AXIS2_PLACEMENT_3D('',#13932,#10909,#10910);
#9514=AXIS2_PLACEMENT_3D('',#13938,#10914,#10915);
#9515=AXIS2_PLACEMENT_3D('',#13940,#10916,#10917);
#9516=AXIS2_PLACEMENT_3D('',#13942,#10919,#10920);
#9517=AXIS2_PLACEMENT_3D('',#13945,#10923,#10924);
#9518=AXIS2_PLACEMENT_3D('',#13947,#10926,#10927);
#9519=AXIS2_PLACEMENT_3D('',#13949,#10929,#10930);
#9520=AXIS2_PLACEMENT_3D('',#13951,#10932,#10933);
#9521=AXIS2_PLACEMENT_3D('',#13953,#10935,#10936);
#9522=AXIS2_PLACEMENT_3D('',#13954,#10937,#10938);
#9523=AXIS2_PLACEMENT_3D('',#13955,#10939,#10940);
#9524=AXIS2_PLACEMENT_3D('',#13957,#10942,#10943);
#9525=AXIS2_PLACEMENT_3D('',#13959,#10945,#10946);
#9526=AXIS2_PLACEMENT_3D('',#13961,#10948,#10949);
#9527=AXIS2_PLACEMENT_3D('',#13963,#10950,#10951);
#9528=AXIS2_PLACEMENT_3D('',#13965,#10953,#10954);
#9529=AXIS2_PLACEMENT_3D('',#13968,#10956,#10957);
#9530=AXIS2_PLACEMENT_3D('',#13969,#10958,#10959);
#9531=AXIS2_PLACEMENT_3D('',#13971,#10960,#10961);
#9532=AXIS2_PLACEMENT_3D('',#13973,#10963,#10964);
#9533=AXIS2_PLACEMENT_3D('',#13976,#10966,#10967);
#9534=AXIS2_PLACEMENT_3D('',#13977,#10968,#10969);
#9535=AXIS2_PLACEMENT_3D('',#13979,#10970,#10971);
#9536=AXIS2_PLACEMENT_3D('',#13981,#10973,#10974);
#9537=AXIS2_PLACEMENT_3D('',#13984,#10976,#10977);
#9538=AXIS2_PLACEMENT_3D('',#13985,#10978,#10979);
#9539=AXIS2_PLACEMENT_3D('',#13987,#10981,#10982);
#9540=AXIS2_PLACEMENT_3D('',#13989,#10984,#10985);
#9541=AXIS2_PLACEMENT_3D('',#13991,#10987,#10988);
#9542=AXIS2_PLACEMENT_3D('',#13993,#10990,#10991);
#9543=AXIS2_PLACEMENT_3D('',#13995,#10993,#10994);
#10794=DIRECTION('axis',(0.,0.,1.));
#10795=DIRECTION('refdir',(1.,0.,0.));
#10796=DIRECTION('center_axis',(-0.707106781186555,-0.70710678118654,0.));
#10797=DIRECTION('ref_axis',(0.,0.,1.));
#10798=DIRECTION('',(0.70710678118654,-0.707106781186555,0.));
#10799=DIRECTION('',(0.,0.,1.));
#10800=DIRECTION('',(-0.70710678118654,0.707106781186555,0.));
#10801=DIRECTION('',(0.,0.,-1.));
#10802=DIRECTION('center_axis',(1.,0.,0.));
#10803=DIRECTION('ref_axis',(0.,-0.707106781186548,-0.707106781186547));
#10804=DIRECTION('',(0.70710678118654,0.,-0.707106781186555));
#10805=DIRECTION('center_axis',(-1.,0.,0.));
#10806=DIRECTION('ref_axis',(0.,-0.707106781186548,-0.707106781186547));
#10807=DIRECTION('center_axis',(1.,0.,0.));
#10808=DIRECTION('ref_axis',(0.,-0.707106781186548,-0.707106781186547));
#10809=DIRECTION('center_axis',(-0.707106781186548,0.,-0.707106781186548));
#10810=DIRECTION('ref_axis',(-0.707106781186548,0.,0.707106781186548));
#10811=DIRECTION('',(0.707106781186548,0.,-0.707106781186548));
#10812=DIRECTION('',(0.,-1.,0.));
#10813=DIRECTION('',(0.,1.,0.));
#10814=DIRECTION('center_axis',(1.,0.,0.));
#10815=DIRECTION('ref_axis',(0.,0.707106781186547,-0.707106781186547));
#10816=DIRECTION('',(0.707106781186532,0.707106781186563,0.));
#10817=DIRECTION('center_axis',(-1.,0.,0.));
#10818=DIRECTION('ref_axis',(0.,0.707106781186548,-0.707106781186548));
#10819=DIRECTION('center_axis',(1.,0.,0.));
#10820=DIRECTION('ref_axis',(0.,0.707106781186547,-0.707106781186547));
#10821=DIRECTION('center_axis',(-0.707106781186555,0.70710678118654,0.));
#10822=DIRECTION('ref_axis',(0.,0.,1.));
#10823=DIRECTION('',(0.70710678118654,0.707106781186555,0.));
#10824=DIRECTION('',(0.,0.,-1.));
#10825=DIRECTION('',(0.,0.,1.));
#10826=DIRECTION('center_axis',(1.,0.,0.));
#10827=DIRECTION('ref_axis',(0.,0.707106781186548,0.707106781186548));
#10828=DIRECTION('',(0.707106781186548,0.,0.707106781186548));
#10829=DIRECTION('center_axis',(-1.,0.,0.));
#10830=DIRECTION('ref_axis',(0.,0.707106781186548,0.707106781186548));
#10831=DIRECTION('center_axis',(1.,0.,0.));
#10832=DIRECTION('ref_axis',(0.,0.707106781186548,0.707106781186548));
#10833=DIRECTION('center_axis',(-0.707106781186532,0.,0.707106781186563));
#10834=DIRECTION('ref_axis',(0.707106781186563,0.,0.707106781186532));
#10835=DIRECTION('',(0.707106781186563,0.,0.707106781186532));
#10836=DIRECTION('',(0.,1.,0.));
#10837=DIRECTION('',(0.,-1.,0.));
#10838=DIRECTION('center_axis',(1.,0.,0.));
#10839=DIRECTION('ref_axis',(0.,-0.707106781186548,0.707106781186548));
#10840=DIRECTION('center_axis',(-1.,0.,0.));
#10841=DIRECTION('ref_axis',(0.,-0.707106781186548,0.707106781186548));
#10842=DIRECTION('center_axis',(1.,0.,0.));
#10843=DIRECTION('ref_axis',(0.,-0.707106781186548,0.707106781186548));
#10844=DIRECTION('center_axis',(1.,0.,0.));
#10845=DIRECTION('ref_axis',(0.,0.707106781186548,0.707106781186548));
#10846=DIRECTION('',(1.,0.,0.));
#10847=DIRECTION('center_axis',(1.,0.,0.));
#10848=DIRECTION('ref_axis',(0.,0.707106781186548,0.707106781186548));
#10849=DIRECTION('',(-1.,0.,0.));
#10850=DIRECTION('center_axis',(0.,0.,1.));
#10851=DIRECTION('ref_axis',(0.,-1.,0.));
#10852=DIRECTION('',(-1.,0.,0.));
#10853=DIRECTION('',(0.,-1.,0.));
#10854=DIRECTION('center_axis',(1.,0.,0.));
#10855=DIRECTION('ref_axis',(0.,-0.707106781186548,0.707106781186548));
#10856=DIRECTION('',(1.,0.,0.));
#10857=DIRECTION('center_axis',(1.,0.,0.));
#10858=DIRECTION('ref_axis',(0.,-0.707106781186548,0.707106781186548));
#10859=DIRECTION('center_axis',(0.,-1.,0.));
#10860=DIRECTION('ref_axis',(0.,0.,-1.));
#10861=DIRECTION('',(-1.,0.,0.));
#10862=DIRECTION('',(0.,0.,-1.));
#10863=DIRECTION('center_axis',(1.,0.,0.));
#10864=DIRECTION('ref_axis',(0.,0.,-1.));
#10865=DIRECTION('center_axis',(1.,0.,0.));
#10866=DIRECTION('ref_axis',(0.,0.,-1.));
#10867=DIRECTION('center_axis',(1.,0.,0.));
#10868=DIRECTION('ref_axis',(0.,0.,-1.));
#10869=DIRECTION('center_axis',(1.,0.,0.));
#10870=DIRECTION('ref_axis',(0.,0.,-1.));
#10871=DIRECTION('center_axis',(1.,0.,0.));
#10872=DIRECTION('ref_axis',(0.,0.,-1.));
#10873=DIRECTION('center_axis',(1.,0.,0.));
#10874=DIRECTION('ref_axis',(0.,0.,-1.));
#10875=DIRECTION('center_axis',(1.,0.,0.));
#10876=DIRECTION('ref_axis',(0.,0.,-1.));
#10877=DIRECTION('center_axis',(-1.,5.71436995156766E-15,0.));
#10878=DIRECTION('ref_axis',(0.,0.,-1.));
#10879=DIRECTION('',(0.382683432365137,1.13142611228768E-16,0.923879532511267));
#10880=DIRECTION('center_axis',(1.,0.,0.));
#10881=DIRECTION('ref_axis',(0.,0.,-1.));
#10882=DIRECTION('center_axis',(1.,0.,0.));
#10883=DIRECTION('ref_axis',(0.,0.,-1.));
#10884=DIRECTION('',(0.,-1.,0.));
#10885=DIRECTION('center_axis',(-1.,0.,0.));
#10886=DIRECTION('ref_axis',(0.,0.707106781186547,-0.707106781186547));
#10887=DIRECTION('',(0.,0.,-1.));
#10888=DIRECTION('center_axis',(-1.,0.,0.));
#10889=DIRECTION('ref_axis',(0.,0.707106781186548,0.707106781186548));
#10890=DIRECTION('',(0.,1.,0.));
#10891=DIRECTION('center_axis',(-1.,0.,0.));
#10892=DIRECTION('ref_axis',(0.,-0.707106781186548,0.707106781186548));
#10893=DIRECTION('',(0.,0.,1.));
#10894=DIRECTION('center_axis',(-1.,0.,0.));
#10895=DIRECTION('ref_axis',(0.,-0.707106781186548,-0.707106781186547));
#10896=DIRECTION('center_axis',(1.,0.,0.));
#10897=DIRECTION('ref_axis',(0.,0.,-1.));
#10898=DIRECTION('center_axis',(-1.,0.,0.));
#10899=DIRECTION('ref_axis',(0.,0.,-1.));
#10900=DIRECTION('center_axis',(1.,0.,0.));
#10901=DIRECTION('ref_axis',(0.,0.,-1.));
#10902=DIRECTION('center_axis',(1.,0.,0.));
#10903=DIRECTION('ref_axis',(0.,0.,-1.));
#10904=DIRECTION('center_axis',(1.,0.,0.));
#10905=DIRECTION('ref_axis',(0.,0.,-1.));
#10906=DIRECTION('',(-0.707106781186545,8.65956056235496E-17,-0.70710678118655));
#10907=DIRECTION('center_axis',(-1.,0.,0.));
#10908=DIRECTION('ref_axis',(0.,0.,-1.));
#10909=DIRECTION('center_axis',(0.707106781186555,0.,-0.70710678118654));
#10910=DIRECTION('ref_axis',(-0.70710678118654,0.,-0.707106781186555));
#10911=DIRECTION('',(0.70710678118654,0.,0.707106781186555));
#10912=DIRECTION('',(-0.70710678118654,0.,-0.707106781186555));
#10913=DIRECTION('',(0.,1.,0.));
#10914=DIRECTION('center_axis',(-1.,0.,0.));
#10915=DIRECTION('ref_axis',(0.,0.707106781186547,-0.707106781186547));
#10916=DIRECTION('center_axis',(1.,0.,0.));
#10917=DIRECTION('ref_axis',(0.,0.707106781186548,-0.707106781186548));
#10918=DIRECTION('',(0.707106781186532,-0.707106781186563,0.));
#10919=DIRECTION('center_axis',(0.707106781186555,0.70710678118654,0.));
#10920=DIRECTION('ref_axis',(0.,0.,-1.));
#10921=DIRECTION('',(0.70710678118654,-0.707106781186555,0.));
#10922=DIRECTION('',(0.,0.,1.));
#10923=DIRECTION('center_axis',(-1.,0.,0.));
#10924=DIRECTION('ref_axis',(0.,0.707106781186548,0.707106781186548));
#10925=DIRECTION('',(0.707106781186548,0.,-0.707106781186548));
#10926=DIRECTION('center_axis',(0.707106781186548,0.,0.707106781186548));
#10927=DIRECTION('ref_axis',(0.707106781186548,0.,-0.707106781186548));
#10928=DIRECTION('',(0.707106781186548,0.,-0.707106781186548));
#10929=DIRECTION('center_axis',(-1.,0.,0.));
#10930=DIRECTION('ref_axis',(0.,-0.707106781186548,0.707106781186548));
#10931=DIRECTION('',(0.707106781186532,0.707106781186563,0.));
#10932=DIRECTION('center_axis',(0.707106781186555,-0.70710678118654,0.));
#10933=DIRECTION('ref_axis',(0.,0.,-1.));
#10934=DIRECTION('',(0.70710678118654,0.707106781186555,0.));
#10935=DIRECTION('center_axis',(-1.,0.,0.));
#10936=DIRECTION('ref_axis',(0.,-0.707106781186548,-0.707106781186547));
#10937=DIRECTION('center_axis',(1.,0.,0.));
#10938=DIRECTION('ref_axis',(0.,-0.707106781186548,-0.707106781186547));
#10939=DIRECTION('center_axis',(0.,1.,0.));
#10940=DIRECTION('ref_axis',(0.,0.,1.));
#10941=DIRECTION('',(1.,0.,0.));
#10942=DIRECTION('center_axis',(1.,0.,0.));
#10943=DIRECTION('ref_axis',(0.,0.707106781186548,-0.707106781186548));
#10944=DIRECTION('',(-1.,0.,0.));
#10945=DIRECTION('center_axis',(0.,0.,-1.));
#10946=DIRECTION('ref_axis',(0.,1.,0.));
#10947=DIRECTION('',(1.,0.,0.));
#10948=DIRECTION('center_axis',(1.,0.,0.));
#10949=DIRECTION('ref_axis',(0.,0.,-1.));
#10950=DIRECTION('center_axis',(-1.,0.,0.));
#10951=DIRECTION('ref_axis',(0.,0.,-1.));
#10952=DIRECTION('',(0.382683432365089,1.1314261122877E-16,0.923879532511287));
#10953=DIRECTION('center_axis',(1.,0.,0.));
#10954=DIRECTION('ref_axis',(0.,0.,-1.));
#10955=DIRECTION('',(-0.707106781186546,8.65956056235495E-17,-0.707106781186548));
#10956=DIRECTION('center_axis',(-1.,0.,0.));
#10957=DIRECTION('ref_axis',(0.,0.,-1.));
#10958=DIRECTION('center_axis',(1.,0.,0.));
#10959=DIRECTION('ref_axis',(0.,0.,-1.));
#10960=DIRECTION('center_axis',(-1.,0.,0.));
#10961=DIRECTION('ref_axis',(0.,0.,-1.));
#10962=DIRECTION('',(0.382683432365089,1.1314261122877E-16,0.923879532511287));
#10963=DIRECTION('center_axis',(1.,0.,0.));
#10964=DIRECTION('ref_axis',(0.,0.,-1.));
#10965=DIRECTION('',(-0.707106781186546,8.65956056235495E-17,-0.707106781186548));
#10966=DIRECTION('center_axis',(-1.,0.,0.));
#10967=DIRECTION('ref_axis',(0.,0.,-1.));
#10968=DIRECTION('center_axis',(1.,0.,0.));
#10969=DIRECTION('ref_axis',(0.,0.,-1.));
#10970=DIRECTION('center_axis',(-1.,5.71436995156766E-15,0.));
#10971=DIRECTION('ref_axis',(0.,0.,-1.));
#10972=DIRECTION('',(0.382683432365137,1.13142611228768E-16,0.923879532511267));
#10973=DIRECTION('center_axis',(1.,0.,0.));
#10974=DIRECTION('ref_axis',(0.,0.,-1.));
#10975=DIRECTION('',(-0.707106781186545,8.65956056235496E-17,-0.70710678118655));
#10976=DIRECTION('center_axis',(-1.,0.,0.));
#10977=DIRECTION('ref_axis',(0.,0.,-1.));
#10978=DIRECTION('center_axis',(-1.,0.,0.));
#10979=DIRECTION('ref_axis',(0.,0.,-1.));
#10980=DIRECTION('',(-1.,0.,0.));
#10981=DIRECTION('center_axis',(-1.,0.,0.));
#10982=DIRECTION('ref_axis',(0.,0.,-1.));
#10983=DIRECTION('',(-1.,0.,0.));
#10984=DIRECTION('center_axis',(-1.,0.,0.));
#10985=DIRECTION('ref_axis',(0.,0.,-1.));
#10986=DIRECTION('',(-1.,0.,0.));
#10987=DIRECTION('center_axis',(-1.,0.,0.));
#10988=DIRECTION('ref_axis',(0.,0.,-1.));
#10989=DIRECTION('',(-1.,0.,0.));
#10990=DIRECTION('center_axis',(-1.,0.,0.));
#10991=DIRECTION('ref_axis',(0.,0.,-1.));
#10992=DIRECTION('',(-1.,0.,0.));
#10993=DIRECTION('center_axis',(1.,0.,0.));
#10994=DIRECTION('ref_axis',(0.,-0.707106781186548,-0.707106781186547));
#13819=CARTESIAN_POINT('',(0.,0.,0.));
#13820=CARTESIAN_POINT('Origin',(100.1,-29.,58.575));
#13821=CARTESIAN_POINT('',(100.,-28.9,26.5));
#13822=CARTESIAN_POINT('',(100.2,-29.1,26.5));
#13823=CARTESIAN_POINT('',(100.,-28.9,26.5));
#13824=CARTESIAN_POINT('',(100.2,-29.1,66.6));
#13825=CARTESIAN_POINT('',(100.2,-29.1,58.575));
#13826=CARTESIAN_POINT('',(100.,-28.9,66.6));
#13827=CARTESIAN_POINT('',(100.2,-29.1,66.6));
#13828=CARTESIAN_POINT('',(100.,-28.9,58.575));
#13829=CARTESIAN_POINT('Origin',(100.1,-25.1,26.5));
#13830=CARTESIAN_POINT('',(100.,-25.1,22.7));
#13831=CARTESIAN_POINT('',(100.2,-25.1,22.5));
#13832=CARTESIAN_POINT('',(100.,-25.1,22.7));
#13833=CARTESIAN_POINT('Origin',(100.2,-25.1,26.5));
#13834=CARTESIAN_POINT('Origin',(100.,-25.1,26.5));
#13835=CARTESIAN_POINT('Origin',(100.1,-14.55,22.6));
#13836=CARTESIAN_POINT('',(100.,25.1,22.7));
#13837=CARTESIAN_POINT('',(100.2,25.1,22.5));
#13838=CARTESIAN_POINT('',(100.,25.1,22.7));
#13839=CARTESIAN_POINT('',(100.2,-14.55,22.5));
#13840=CARTESIAN_POINT('',(100.,-14.55,22.7));
#13841=CARTESIAN_POINT('Origin',(100.1,25.1,26.5));
#13842=CARTESIAN_POINT('',(100.,28.9,26.5));
#13843=CARTESIAN_POINT('',(100.2,29.1,26.5));
#13844=CARTESIAN_POINT('',(100.,28.9,26.5));
#13845=CARTESIAN_POINT('Origin',(100.2,25.1,26.5));
#13846=CARTESIAN_POINT('Origin',(100.,25.1,26.5));
#13847=CARTESIAN_POINT('Origin',(100.1,29.,34.525));
#13848=CARTESIAN_POINT('',(100.,28.9,66.6));
#13849=CARTESIAN_POINT('',(100.2,29.1,66.6));
#13850=CARTESIAN_POINT('',(100.,28.9,66.6));
#13851=CARTESIAN_POINT('',(100.2,29.1,34.525));
#13852=CARTESIAN_POINT('',(100.,28.9,34.525));
#13853=CARTESIAN_POINT('Origin',(100.1,25.1,66.6));
#13854=CARTESIAN_POINT('',(100.,25.1,70.4));
#13855=CARTESIAN_POINT('',(100.2,25.1,70.6));
#13856=CARTESIAN_POINT('',(100.,25.1,70.4));
#13857=CARTESIAN_POINT('Origin',(100.2,25.1,66.6));
#13858=CARTESIAN_POINT('Origin',(100.,25.1,66.6));
#13859=CARTESIAN_POINT('Origin',(100.1,14.55,70.5));
#13860=CARTESIAN_POINT('',(100.,-25.1,70.4));
#13861=CARTESIAN_POINT('',(100.2,-25.1,70.6));
#13862=CARTESIAN_POINT('',(100.,-25.1,70.4));
#13863=CARTESIAN_POINT('',(100.2,14.55,70.6));
#13864=CARTESIAN_POINT('',(100.,14.55,70.4));
#13865=CARTESIAN_POINT('Origin',(100.1,-25.1,66.6));
#13866=CARTESIAN_POINT('Origin',(100.2,-25.1,66.6));
#13867=CARTESIAN_POINT('Origin',(100.,-25.1,66.6));
#13868=CARTESIAN_POINT('Origin',(100.,25.1,66.6));
#13869=CARTESIAN_POINT('',(102.8,25.1,70.6));
#13870=CARTESIAN_POINT('',(100.,25.1,70.6));
#13871=CARTESIAN_POINT('',(102.8,29.1,66.6));
#13872=CARTESIAN_POINT('Origin',(102.8,25.1,66.6));
#13873=CARTESIAN_POINT('',(100.,29.1,66.6));
#13874=CARTESIAN_POINT('Origin',(100.,29.1,70.6));
#13875=CARTESIAN_POINT('',(102.8,-25.1,70.6));
#13876=CARTESIAN_POINT('',(100.,-25.1,70.6));
#13877=CARTESIAN_POINT('',(102.8,14.55,70.6));
#13878=CARTESIAN_POINT('Origin',(100.,-25.1,66.6));
#13879=CARTESIAN_POINT('',(102.8,-29.1,66.6));
#13880=CARTESIAN_POINT('',(100.,-29.1,66.6));
#13881=CARTESIAN_POINT('Origin',(102.8,-25.1,66.6));
#13882=CARTESIAN_POINT('Origin',(100.,-29.1,70.6));
#13883=CARTESIAN_POINT('',(102.8,-29.1,26.5));
#13884=CARTESIAN_POINT('',(100.,-29.1,26.5));
#13885=CARTESIAN_POINT('',(102.8,-29.1,58.575));
#13886=CARTESIAN_POINT('Origin',(100.,0.,46.55));
#13887=CARTESIAN_POINT('',(100.,25.,28.2));
#13888=CARTESIAN_POINT('Origin',(100.,25.,26.5));
#13889=CARTESIAN_POINT('',(100.,-25.,68.2));
#13890=CARTESIAN_POINT('Origin',(100.,-25.,66.5));
#13891=CARTESIAN_POINT('',(100.,-25.,28.2));
#13892=CARTESIAN_POINT('Origin',(100.,-25.,26.5));
#13893=CARTESIAN_POINT('',(100.,25.,68.2));
#13894=CARTESIAN_POINT('Origin',(100.,25.,66.5));
#13895=CARTESIAN_POINT('',(100.,-7.9602041944578E-16,54.));
#13896=CARTESIAN_POINT('Origin',(100.,0.,47.5));
#13897=CARTESIAN_POINT('Origin',(102.929289321881,-25.,66.5));
#13898=CARTESIAN_POINT('',(102.858578643763,-25.,69.6085786437627));
#13899=CARTESIAN_POINT('Origin',(102.858578643763,-25.,66.5));
#13900=CARTESIAN_POINT('',(103.,-25.,69.95));
#13901=CARTESIAN_POINT('',(102.929289321881,-25.,69.7792893218814));
#13902=CARTESIAN_POINT('Origin',(103.,-25.,66.5));
#13903=CARTESIAN_POINT('Origin',(103.,0.,46.55));
#13904=CARTESIAN_POINT('',(103.,25.1,22.7));
#13905=CARTESIAN_POINT('',(103.,-25.1,22.7));
#13906=CARTESIAN_POINT('',(103.,-14.55,22.7));
#13907=CARTESIAN_POINT('',(103.,28.9,26.5));
#13908=CARTESIAN_POINT('Origin',(103.,25.1,26.5));
#13909=CARTESIAN_POINT('',(103.,28.9,66.6));
#13910=CARTESIAN_POINT('',(103.,28.9,34.525));
#13911=CARTESIAN_POINT('',(103.,25.1,70.4));
#13912=CARTESIAN_POINT('Origin',(103.,25.1,66.6));
#13913=CARTESIAN_POINT('',(103.,-25.1,70.4));
#13914=CARTESIAN_POINT('',(103.,14.55,70.4));
#13915=CARTESIAN_POINT('',(103.,-28.9,66.6));
#13916=CARTESIAN_POINT('Origin',(103.,-25.1,66.6));
#13917=CARTESIAN_POINT('',(103.,-28.9,26.5));
#13918=CARTESIAN_POINT('',(103.,-28.9,58.575));
#13919=CARTESIAN_POINT('Origin',(103.,-25.1,26.5));
#13920=CARTESIAN_POINT('',(103.,-25.,29.95));
#13921=CARTESIAN_POINT('Origin',(103.,-25.,26.5));
#13922=CARTESIAN_POINT('',(103.,-7.9602041944578E-16,54.));
#13923=CARTESIAN_POINT('Origin',(103.,0.,47.5));
#13924=CARTESIAN_POINT('',(103.,25.,69.95));
#13925=CARTESIAN_POINT('Origin',(103.,25.,66.5));
#13926=CARTESIAN_POINT('',(103.,25.,29.95));
#13927=CARTESIAN_POINT('Origin',(103.,25.,26.5));
#13928=CARTESIAN_POINT('Origin',(102.225,-25.,66.5));
#13929=CARTESIAN_POINT('',(101.45,-25.,68.2));
#13930=CARTESIAN_POINT('',(102.225,-25.,68.975));
#13931=CARTESIAN_POINT('Origin',(101.45,-25.,66.5));
#13932=CARTESIAN_POINT('Origin',(102.9,-14.55,22.6));
#13933=CARTESIAN_POINT('',(102.8,25.1,22.5));
#13934=CARTESIAN_POINT('',(102.8,25.1,22.5));
#13935=CARTESIAN_POINT('',(102.8,-25.1,22.5));
#13936=CARTESIAN_POINT('',(103.,-25.1,22.7));
#13937=CARTESIAN_POINT('',(102.8,-14.55,22.5));
#13938=CARTESIAN_POINT('Origin',(102.9,25.1,26.5));
#13939=CARTESIAN_POINT('',(102.8,29.1,26.5));
#13940=CARTESIAN_POINT('Origin',(102.8,25.1,26.5));
#13941=CARTESIAN_POINT('',(102.8,29.1,26.5));
#13942=CARTESIAN_POINT('Origin',(102.9,29.,34.525));
#13943=CARTESIAN_POINT('',(102.8,29.1,66.6));
#13944=CARTESIAN_POINT('',(102.8,29.1,34.525));
#13945=CARTESIAN_POINT('Origin',(102.9,25.1,66.6));
#13946=CARTESIAN_POINT('',(102.8,25.1,70.6));
#13947=CARTESIAN_POINT('Origin',(102.9,14.55,70.5));
#13948=CARTESIAN_POINT('',(102.8,-25.1,70.6));
#13949=CARTESIAN_POINT('Origin',(102.9,-25.1,66.6));
#13950=CARTESIAN_POINT('',(102.8,-29.1,66.6));
#13951=CARTESIAN_POINT('Origin',(102.9,-29.,58.575));
#13952=CARTESIAN_POINT('',(102.8,-29.1,26.5));
#13953=CARTESIAN_POINT('Origin',(102.9,-25.1,26.5));
#13954=CARTESIAN_POINT('Origin',(102.8,-25.1,26.5));
#13955=CARTESIAN_POINT('Origin',(100.,29.1,22.5));
#13956=CARTESIAN_POINT('',(100.,29.1,26.5));
#13957=CARTESIAN_POINT('Origin',(100.,25.1,26.5));
#13958=CARTESIAN_POINT('',(100.,25.1,22.5));
#13959=CARTESIAN_POINT('Origin',(100.,-29.1,22.5));
#13960=CARTESIAN_POINT('',(100.,-25.1,22.5));
#13961=CARTESIAN_POINT('Origin',(102.929289321881,25.,26.5));
#13962=CARTESIAN_POINT('',(102.858578643763,25.,29.6085786437627));
#13963=CARTESIAN_POINT('Origin',(102.858578643763,25.,26.5));
#13964=CARTESIAN_POINT('',(102.929289321881,25.,29.7792893218814));
#13965=CARTESIAN_POINT('Origin',(102.225,25.,26.5));
#13966=CARTESIAN_POINT('',(101.45,25.,28.2));
#13967=CARTESIAN_POINT('',(102.225,25.,28.975));
#13968=CARTESIAN_POINT('Origin',(101.45,25.,26.5));
#13969=CARTESIAN_POINT('Origin',(102.929289321881,-25.,26.5));
#13970=CARTESIAN_POINT('',(102.858578643763,-25.,29.6085786437627));
#13971=CARTESIAN_POINT('Origin',(102.858578643763,-25.,26.5));
#13972=CARTESIAN_POINT('',(102.929289321881,-25.,29.7792893218814));
#13973=CARTESIAN_POINT('Origin',(102.225,-25.,26.5));
#13974=CARTESIAN_POINT('',(101.45,-25.,28.2));
#13975=CARTESIAN_POINT('',(102.225,-25.,28.975));
#13976=CARTESIAN_POINT('Origin',(101.45,-25.,26.5));
#13977=CARTESIAN_POINT('Origin',(102.929289321881,25.,66.5));
#13978=CARTESIAN_POINT('',(102.858578643763,25.,69.6085786437627));
#13979=CARTESIAN_POINT('Origin',(102.858578643763,25.,66.5));
#13980=CARTESIAN_POINT('',(102.929289321881,25.,69.7792893218814));
#13981=CARTESIAN_POINT('Origin',(102.225,25.,66.5));
#13982=CARTESIAN_POINT('',(101.45,25.,68.2));
#13983=CARTESIAN_POINT('',(102.225,25.,68.975));
#13984=CARTESIAN_POINT('Origin',(101.45,25.,66.5));
#13985=CARTESIAN_POINT('Origin',(103.,25.,66.5));
#13986=CARTESIAN_POINT('',(103.,25.,68.2));
#13987=CARTESIAN_POINT('Origin',(103.,-25.,26.5));
#13988=CARTESIAN_POINT('',(103.,-25.,28.2));
#13989=CARTESIAN_POINT('Origin',(103.,-25.,66.5));
#13990=CARTESIAN_POINT('',(103.,-25.,68.2));
#13991=CARTESIAN_POINT('Origin',(103.,25.,26.5));
#13992=CARTESIAN_POINT('',(103.,25.,28.2));
#13993=CARTESIAN_POINT('Origin',(103.,0.,47.5));
#13994=CARTESIAN_POINT('',(103.,7.9602041944578E-16,54.));
#13995=CARTESIAN_POINT('Origin',(100.,-25.1,26.5));
#18256=UNCERTAINTY_MEASURE_WITH_UNIT(LENGTH_MEASURE(0.01),#18282,
'DISTANCE_ACCURACY_VALUE',
'Maximum model space distance between geometric entities at asserted c
onnectivities');
#18266=UNCERTAINTY_MEASURE_WITH_UNIT(LENGTH_MEASURE(0.01),#18282,
'DISTANCE_ACCURACY_VALUE',
'Maximum model space distance between geometric entities at asserted c
onnectivities');
#18271=(
GEOMETRIC_REPRESENTATION_CONTEXT(3)
GLOBAL_UNCERTAINTY_ASSIGNED_CONTEXT((#18256))
GLOBAL_UNIT_ASSIGNED_CONTEXT((#18282,#18284,#18285))
REPRESENTATION_CONTEXT('','3D')
);
#18281=(
GEOMETRIC_REPRESENTATION_CONTEXT(3)
GLOBAL_UNCERTAINTY_ASSIGNED_CONTEXT((#18266))
GLOBAL_UNIT_ASSIGNED_CONTEXT((#18282,#18284,#18285))
REPRESENTATION_CONTEXT('','3D')
);
#18282=(
LENGTH_UNIT()
NAMED_UNIT(*)
SI_UNIT(.MILLI.,.METRE.)
);
#18284=(
NAMED_UNIT(*)
PLANE_ANGLE_UNIT()
SI_UNIT($,.RADIAN.)
);
#18285=(
NAMED_UNIT(*)
SI_UNIT($,.STERADIAN.)
SOLID_ANGLE_UNIT()
);
#18290=SHAPE_DEFINITION_REPRESENTATION(#18304,#18342);
#18304=PRODUCT_DEFINITION_SHAPE('',$,#18357);
#18342=SHAPE_REPRESENTATION('',(#9470),#18271);
#18352=PRODUCT_DEFINITION_CONTEXT('part definition',#18396,'design');
#18357=PRODUCT_DEFINITION('2026-10-20-13-03-21-308',
'07_Rear_Cover_Plate',#18371,#18352);
#18371=PRODUCT_DEFINITION_FORMATION('',$,#18402);
#18396=APPLICATION_CONTEXT(
'Core Data for Automotive Mechanical Design Process');
#18397=PRODUCT_CONTEXT('part definition',#18396,'mechanical');
#18402=PRODUCT('2026-10-20-13-03-21-308','07_Rear_Cover_Plate',$,(#18397));
#18461=COLOUR_RGB('Sky Blue',0.24,0.69,0.87);
#18462=FILL_AREA_STYLE_COLOUR('',#18461);
#18463=FILL_AREA_STYLE('',(#18462));
#18464=SURFACE_STYLE_FILL_AREA(#18463);
#18465=SURFACE_SIDE_STYLE('',(#18464));
#18466=SURFACE_STYLE_USAGE(.BOTH.,#18465);
#18467=PRESENTATION_STYLE_ASSIGNMENT((#18466));
ENDSEC;
END-ISO-10303-21;
